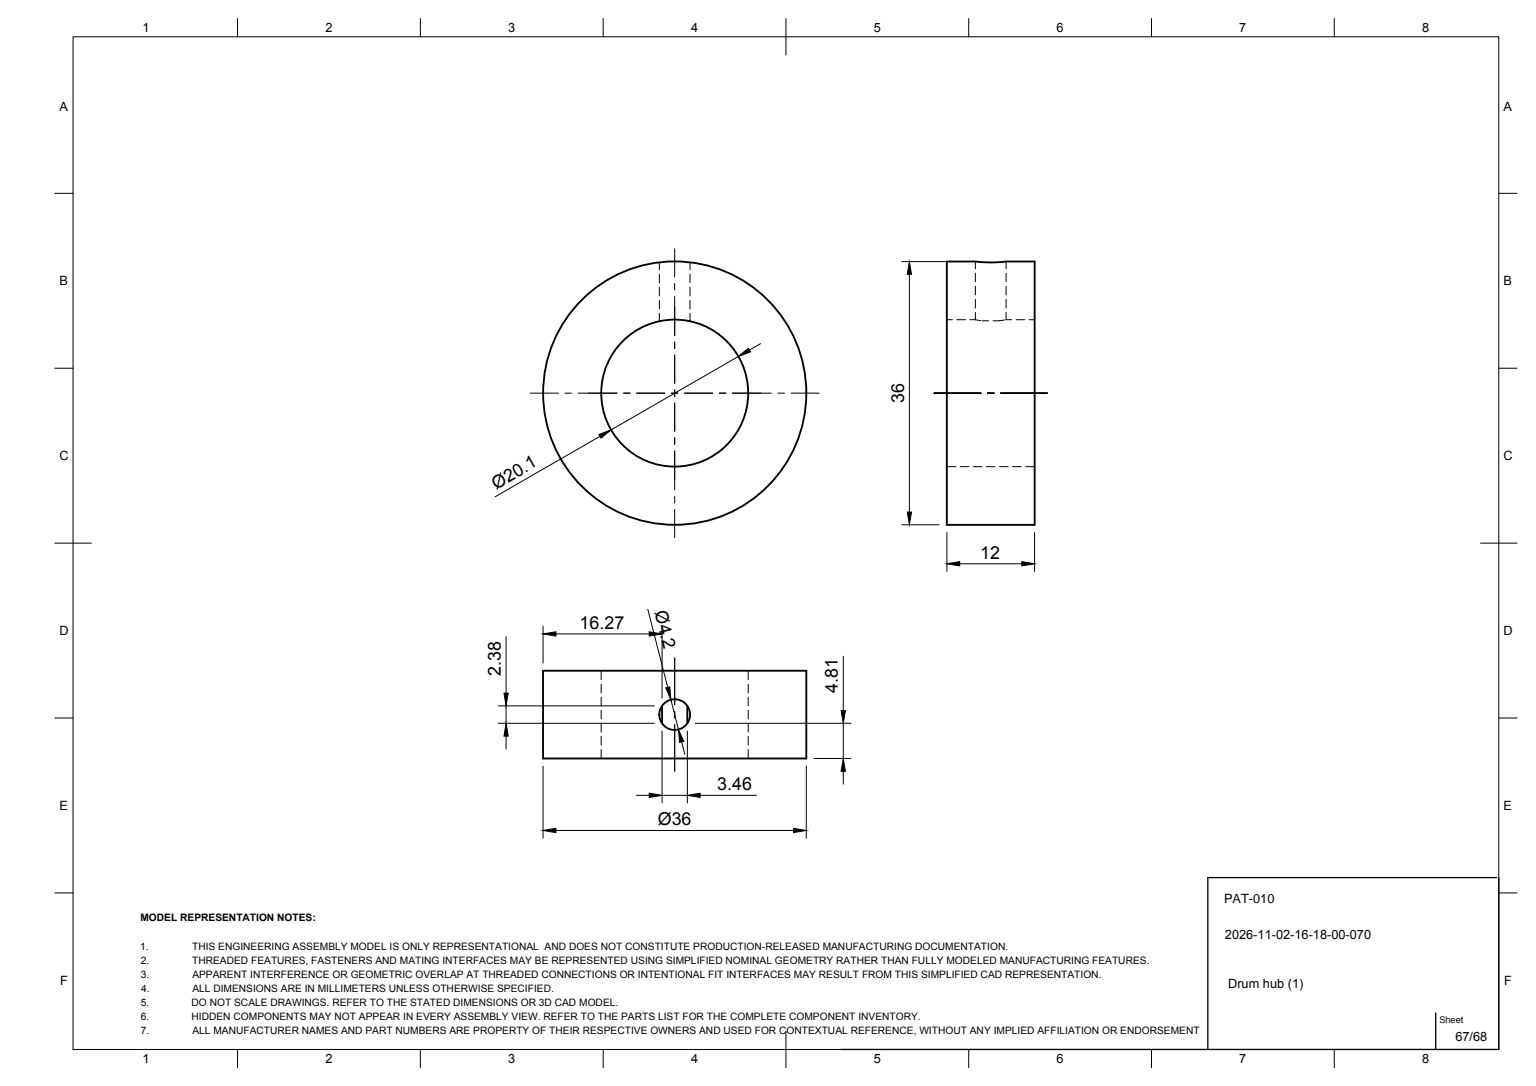
ISO-10303-21;
HEADER;
/* Generated by software containing ST-Developer
 * from STEP Tools, Inc. (www.steptools.com) 
 */

FILE_DESCRIPTION(
/* description */ ('Belt conveyor head drive unit'),
/* implementation_level */ '2;1');

FILE_NAME(
/* name */ 'Drum hub (1).step',
/* time_stamp */ '2026-10-28T03:26:19-07:00',
/* author */ (''),
/* organization */ (''),
/* preprocessor_version */ 'ST-DEVELOPER v20.2',
/* originating_system */ 'Autodesk Translation Framework v15.17.0.0',
/* authorisation */ '');

FILE_SCHEMA (('AUTOMOTIVE_DESIGN { 1 0 10303 214 3 1 1 }'));
ENDSEC;

DATA;
#10=MECHANICAL_DESIGN_GEOMETRIC_PRESENTATION_REPRESENTATION('',(#928),#27069);
#619=B_SPLINE_CURVE_WITH_KNOTS('',3,(#25750,#25751,#25752,#25753,#25754,
#25755,#25756,#25757,#25758,#25759,#25760,#25761,#25762,#25763),
 .UNSPECIFIED.,.F.,.F.,(4,2,2,2,2,2,4),(0.756005737987017,0.793568827564644,
0.872922520054199,0.952276212543754,1.03162990503331,1.11098359752286,1.1485466871005),
 .UNSPECIFIED.);
#620=B_SPLINE_CURVE_WITH_KNOTS('',3,(#25769,#25770,#25771,#25772,#25773,
#25774,#25775,#25776,#25777,#25778,#25779,#25780,#25781,#25782,#25783,#25784,
#25785,#25786),.UNSPECIFIED.,.F.,.F.,(4,2,2,2,2,2,2,2,4),(0.,0.0791819055472362,
0.158363811094472,0.237545215630595,0.316726620166717,0.395908024702839,
0.475089429238961,0.554271334786197,0.633453240333433),.UNSPECIFIED.);
#621=B_SPLINE_CURVE_WITH_KNOTS('',3,(#25787,#25788,#25789,#25790,#25791,
#25792,#25793,#25794,#25795,#25796,#25797,#25798,#25799,#25800,#25801,#25802,
#25803,#25804),.UNSPECIFIED.,.F.,.F.,(4,2,2,2,2,2,2,2,4),(0.633453240333433,
0.71263514588067,0.791817051427906,0.870998455964028,0.95017986050015,1.02936126503627,
1.10854266957239,1.18772457511963,1.26690648066687),.UNSPECIFIED.);
#622=B_SPLINE_CURVE_WITH_KNOTS('',3,(#25807,#25808,#25809,#25810,#25811,
#25812,#25813,#25814,#25815,#25816,#25817,#25818,#25819,#25820),
 .UNSPECIFIED.,.F.,.F.,(4,2,2,2,2,2,4),(0.121154929624508,0.158718019202141,
0.238071711691696,0.317425404181251,0.396779096670806,0.476132789160361,
0.513695878737978),.UNSPECIFIED.);
#774=SHAPE_REPRESENTATION_RELATIONSHIP('SRR','None',#27423,#843);
#843=ADVANCED_BREP_SHAPE_REPRESENTATION('',(#1009),#27065);
#928=STYLED_ITEM('',(#27783),#1009);
#1009=MANIFOLD_SOLID_BREP('Body1',#13797);
#1260=FACE_BOUND('',#3356,.T.);
#1261=FACE_BOUND('',#3358,.T.);
#1262=FACE_BOUND('',#3360,.T.);
#1263=FACE_BOUND('',#3362,.T.);
#1604=PLANE('',#16002);
#1605=PLANE('',#16007);
#1606=PLANE('',#16014);
#1607=PLANE('',#16015);
#2304=FACE_OUTER_BOUND('',#3352,.T.);
#2305=FACE_OUTER_BOUND('',#3353,.T.);
#2306=FACE_OUTER_BOUND('',#3354,.T.);
#2307=FACE_OUTER_BOUND('',#3355,.T.);
#2308=FACE_OUTER_BOUND('',#3357,.T.);
#2309=FACE_OUTER_BOUND('',#3359,.T.);
#2310=FACE_OUTER_BOUND('',#3361,.T.);
#3352=EDGE_LOOP('',(#11826,#11827));
#3353=EDGE_LOOP('',(#11828,#11829,#11830,#11831,#11832,#11833,#11834,#11835,
#11836));
#3354=EDGE_LOOP('',(#11837,#11838,#11839));
#3355=EDGE_LOOP('',(#11840,#11841,#11842,#11843));
#3356=EDGE_LOOP('',(#11844,#11845,#11846,#11847));
#3357=EDGE_LOOP('',(#11848,#11849,#11850,#11851));
#3358=EDGE_LOOP('',(#11852,#11853));
#3359=EDGE_LOOP('',(#11854));
#3360=EDGE_LOOP('',(#11855));
#3361=EDGE_LOOP('',(#11856));
#3362=EDGE_LOOP('',(#11857));
#4150=LINE('',#25746,#4942);
#4151=LINE('',#25767,#4943);
#4152=LINE('',#25822,#4944);
#4153=LINE('',#25827,#4945);
#4154=LINE('',#25833,#4946);
#4942=VECTOR('',#19968,1.);
#4943=VECTOR('',#19975,0.21);
#4944=VECTOR('',#19980,1.);
#4945=VECTOR('',#19985,1.005);
#4946=VECTOR('',#19992,1.8);
#5766=CIRCLE('',#16003,0.21);
#5767=CIRCLE('',#16005,0.21);
#5768=CIRCLE('',#16006,0.21);
#5769=CIRCLE('',#16009,1.005);
#5770=CIRCLE('',#16010,1.005);
#5771=CIRCLE('',#16012,1.8);
#5772=CIRCLE('',#16013,1.8);
#6934=VERTEX_POINT('',#25744);
#6935=VERTEX_POINT('',#25745);
#6936=VERTEX_POINT('',#25749);
#6937=VERTEX_POINT('',#25764);
#6938=VERTEX_POINT('',#25766);
#6939=VERTEX_POINT('',#25768);
#6940=VERTEX_POINT('',#25805);
#6941=VERTEX_POINT('',#25824);
#6942=VERTEX_POINT('',#25826);
#6943=VERTEX_POINT('',#25830);
#6944=VERTEX_POINT('',#25832);
#8605=EDGE_CURVE('',#6934,#6935,#4150,.T.);
#8606=EDGE_CURVE('',#6934,#6935,#5766,.T.);
#8607=EDGE_CURVE('',#6936,#6934,#619,.T.);
#8608=EDGE_CURVE('',#6937,#6936,#5767,.T.);
#8609=EDGE_CURVE('',#6937,#6938,#4151,.T.);
#8610=EDGE_CURVE('',#6939,#6938,#620,.T.);
#8611=EDGE_CURVE('',#6938,#6939,#621,.T.);
#8612=EDGE_CURVE('',#6940,#6937,#5768,.T.);
#8613=EDGE_CURVE('',#6935,#6940,#622,.T.);
#8614=EDGE_CURVE('',#6940,#6936,#4152,.T.);
#8615=EDGE_CURVE('',#6941,#6941,#5769,.T.);
#8616=EDGE_CURVE('',#6941,#6942,#4153,.T.);
#8617=EDGE_CURVE('',#6942,#6942,#5770,.T.);
#8618=EDGE_CURVE('',#6943,#6943,#5771,.T.);
#8619=EDGE_CURVE('',#6943,#6944,#4154,.T.);
#8620=EDGE_CURVE('',#6944,#6944,#5772,.T.);
#11826=ORIENTED_EDGE('',*,*,#8605,.F.);
#11827=ORIENTED_EDGE('',*,*,#8606,.T.);
#11828=ORIENTED_EDGE('',*,*,#8607,.F.);
#11829=ORIENTED_EDGE('',*,*,#8608,.F.);
#11830=ORIENTED_EDGE('',*,*,#8609,.T.);
#11831=ORIENTED_EDGE('',*,*,#8610,.F.);
#11832=ORIENTED_EDGE('',*,*,#8611,.F.);
#11833=ORIENTED_EDGE('',*,*,#8609,.F.);
#11834=ORIENTED_EDGE('',*,*,#8612,.F.);
#11835=ORIENTED_EDGE('',*,*,#8613,.F.);
#11836=ORIENTED_EDGE('',*,*,#8606,.F.);
#11837=ORIENTED_EDGE('',*,*,#8614,.F.);
#11838=ORIENTED_EDGE('',*,*,#8612,.T.);
#11839=ORIENTED_EDGE('',*,*,#8608,.T.);
#11840=ORIENTED_EDGE('',*,*,#8615,.F.);
#11841=ORIENTED_EDGE('',*,*,#8616,.T.);
#11842=ORIENTED_EDGE('',*,*,#8617,.T.);
#11843=ORIENTED_EDGE('',*,*,#8616,.F.);
#11844=ORIENTED_EDGE('',*,*,#8613,.T.);
#11845=ORIENTED_EDGE('',*,*,#8614,.T.);
#11846=ORIENTED_EDGE('',*,*,#8607,.T.);
#11847=ORIENTED_EDGE('',*,*,#8605,.T.);
#11848=ORIENTED_EDGE('',*,*,#8618,.F.);
#11849=ORIENTED_EDGE('',*,*,#8619,.T.);
#11850=ORIENTED_EDGE('',*,*,#8620,.T.);
#11851=ORIENTED_EDGE('',*,*,#8619,.F.);
#11852=ORIENTED_EDGE('',*,*,#8610,.T.);
#11853=ORIENTED_EDGE('',*,*,#8611,.T.);
#11854=ORIENTED_EDGE('',*,*,#8618,.T.);
#11855=ORIENTED_EDGE('',*,*,#8615,.T.);
#11856=ORIENTED_EDGE('',*,*,#8620,.F.);
#11857=ORIENTED_EDGE('',*,*,#8617,.F.);
#12818=CYLINDRICAL_SURFACE('',#16004,0.21);
#12819=CYLINDRICAL_SURFACE('',#16008,1.005);
#12820=CYLINDRICAL_SURFACE('',#16011,1.8);
#13583=ADVANCED_FACE('',(#2304),#1604,.T.);
#13584=ADVANCED_FACE('',(#2305),#12818,.F.);
#13585=ADVANCED_FACE('',(#2306),#1605,.T.);
#13586=ADVANCED_FACE('',(#2307,#1260),#12819,.F.);
#13587=ADVANCED_FACE('',(#2308,#1261),#12820,.T.);
#13588=ADVANCED_FACE('',(#2309,#1262),#1606,.T.);
#13589=ADVANCED_FACE('',(#2310,#1263),#1607,.F.);
#13797=CLOSED_SHELL('',(#13583,#13584,#13585,#13586,#13587,#13588,#13589));
#16001=AXIS2_PLACEMENT_3D('',#25742,#19964,#19965);
#16002=AXIS2_PLACEMENT_3D('',#25743,#19966,#19967);
#16003=AXIS2_PLACEMENT_3D('',#25747,#19969,#19970);
#16004=AXIS2_PLACEMENT_3D('',#25748,#19971,#19972);
#16005=AXIS2_PLACEMENT_3D('',#25765,#19973,#19974);
#16006=AXIS2_PLACEMENT_3D('',#25806,#19976,#19977);
#16007=AXIS2_PLACEMENT_3D('',#25821,#19978,#19979);
#16008=AXIS2_PLACEMENT_3D('',#25823,#19981,#19982);
#16009=AXIS2_PLACEMENT_3D('',#25825,#19983,#19984);
#16010=AXIS2_PLACEMENT_3D('',#25828,#19986,#19987);
#16011=AXIS2_PLACEMENT_3D('',#25829,#19988,#19989);
#16012=AXIS2_PLACEMENT_3D('',#25831,#19990,#19991);
#16013=AXIS2_PLACEMENT_3D('',#25834,#19993,#19994);
#16014=AXIS2_PLACEMENT_3D('',#25835,#19995,#19996);
#16015=AXIS2_PLACEMENT_3D('',#25836,#19997,#19998);
#19964=DIRECTION('axis',(0.,0.,1.));
#19965=DIRECTION('refdir',(1.,0.,0.));
#19966=DIRECTION('center_axis',(0.,0.,1.));
#19967=DIRECTION('ref_axis',(1.,0.,0.));
#19968=DIRECTION('',(0.,1.,0.));
#19969=DIRECTION('center_axis',(0.,0.,1.));
#19970=DIRECTION('ref_axis',(1.,0.,0.));
#19971=DIRECTION('center_axis',(0.,0.,1.));
#19972=DIRECTION('ref_axis',(1.,0.,0.));
#19973=DIRECTION('center_axis',(0.,0.,1.));
#19974=DIRECTION('ref_axis',(1.,0.,0.));
#19975=DIRECTION('',(0.,0.,1.));
#19976=DIRECTION('center_axis',(0.,0.,1.));
#19977=DIRECTION('ref_axis',(1.,0.,0.));
#19978=DIRECTION('center_axis',(0.,0.,1.));
#19979=DIRECTION('ref_axis',(1.,0.,0.));
#19980=DIRECTION('',(0.,-1.,0.));
#19981=DIRECTION('center_axis',(0.,1.,0.));
#19982=DIRECTION('ref_axis',(1.,0.,0.));
#19983=DIRECTION('center_axis',(0.,-1.,0.));
#19984=DIRECTION('ref_axis',(1.,0.,0.));
#19985=DIRECTION('',(0.,-1.,0.));
#19986=DIRECTION('center_axis',(0.,-1.,0.));
#19987=DIRECTION('ref_axis',(1.,0.,0.));
#19988=DIRECTION('center_axis',(0.,1.,0.));
#19989=DIRECTION('ref_axis',(1.,0.,0.));
#19990=DIRECTION('center_axis',(0.,1.,0.));
#19991=DIRECTION('ref_axis',(1.,0.,0.));
#19992=DIRECTION('',(0.,-1.,0.));
#19993=DIRECTION('center_axis',(0.,1.,0.));
#19994=DIRECTION('ref_axis',(1.,0.,0.));
#19995=DIRECTION('center_axis',(0.,1.,0.));
#19996=DIRECTION('ref_axis',(1.,0.,0.));
#19997=DIRECTION('center_axis',(0.,1.,0.));
#19998=DIRECTION('ref_axis',(1.,0.,0.));
#25742=CARTESIAN_POINT('',(0.,0.,0.));
#25743=CARTESIAN_POINT('Origin',(6.97091003018116,36.4,7.99));
#25744=CARTESIAN_POINT('',(7.14389846910121,36.2809411910021,7.99));
#25745=CARTESIAN_POINT('',(7.14389846910121,36.5190588089979,7.99));
#25746=CARTESIAN_POINT('',(7.14389846910121,35.8,7.99));
#25747=CARTESIAN_POINT('Origin',(6.97091003018116,36.4,7.99));
#25748=CARTESIAN_POINT('Origin',(6.97091003018116,36.4,7.99));
#25749=CARTESIAN_POINT('',(6.7979215912611,36.2809411910021,7.99));
#25750=CARTESIAN_POINT('Ctrl Pts',(6.7979215912611,36.2809411910021,7.99));
#25751=CARTESIAN_POINT('Ctrl Pts',(6.80531516486984,36.2701985776047,7.99129192197638));
#25752=CARTESIAN_POINT('Ctrl Pts',(6.81361289145555,36.2603122906273,7.99265394943905));
#25753=CARTESIAN_POINT('Ctrl Pts',(6.84101795633608,36.2329072257467,7.9967480843909));
#25754=CARTESIAN_POINT('Ctrl Pts',(6.86457986242187,36.216757943667,7.99969589327637));
#25755=CARTESIAN_POINT('Ctrl Pts',(6.91629712554875,36.1953022060351,8.00385029472357));
#25756=CARTESIAN_POINT('Ctrl Pts',(6.9444587993513,36.19,8.005));
#25757=CARTESIAN_POINT('Ctrl Pts',(6.99736126101101,36.19,8.005));
#25758=CARTESIAN_POINT('Ctrl Pts',(7.02552293481357,36.1953022060351,8.00385029472357));
#25759=CARTESIAN_POINT('Ctrl Pts',(7.07724019794044,36.216757943667,7.99969589327637));
#25760=CARTESIAN_POINT('Ctrl Pts',(7.10080210402623,36.2329072257467,7.9967480843909));
#25761=CARTESIAN_POINT('Ctrl Pts',(7.12820716890676,36.2603122906273,7.99265394943905));
#25762=CARTESIAN_POINT('Ctrl Pts',(7.13650489549247,36.2701985776047,7.99129192197638));
#25763=CARTESIAN_POINT('Ctrl Pts',(7.14389846910121,36.2809411910021,7.99));
#25764=CARTESIAN_POINT('',(6.76091003018116,36.4,7.99));
#25765=CARTESIAN_POINT('Origin',(6.97091003018116,36.4,7.99));
#25766=CARTESIAN_POINT('',(6.76091003018116,36.4,8.78770802985275));
#25767=CARTESIAN_POINT('',(6.76091003018116,36.4,7.99));
#25768=CARTESIAN_POINT('',(7.18091003018116,36.4,8.78770802985275));
#25769=CARTESIAN_POINT('Ctrl Pts',(7.18091003018116,36.4,8.78770802985275));
#25770=CARTESIAN_POINT('Ctrl Pts',(7.18091003018116,36.3736060314843,8.78770802985275));
#25771=CARTESIAN_POINT('Ctrl Pts',(7.17563026313289,36.345469345566,8.78835284034214));
#25772=CARTESIAN_POINT('Ctrl Pts',(7.15419155416006,36.293736883974,8.79067700538683));
#25773=CARTESIAN_POINT('Ctrl Pts',(7.13803391906352,36.270139040784,8.79232226897314));
#25774=CARTESIAN_POINT('Ctrl Pts',(7.10077110728482,36.2328762290053,8.79540680803063));
#25775=CARTESIAN_POINT('Ctrl Pts',(7.07717321270923,36.2167185016358,8.79704717240673));
#25776=CARTESIAN_POINT('Ctrl Pts',(7.02544057769236,36.1952797246826,8.79936011492601));
#25777=CARTESIAN_POINT('Ctrl Pts',(6.9973038316932,36.19,8.8));
#25778=CARTESIAN_POINT('Ctrl Pts',(6.94451622866912,36.19,8.8));
#25779=CARTESIAN_POINT('Ctrl Pts',(6.91637948266995,36.1952797246826,8.79936011492601));
#25780=CARTESIAN_POINT('Ctrl Pts',(6.86464684765309,36.2167185016358,8.79704717240673));
#25781=CARTESIAN_POINT('Ctrl Pts',(6.84104895307749,36.2328762290053,8.79540680803063));
#25782=CARTESIAN_POINT('Ctrl Pts',(6.80378614129879,36.270139040784,8.79232226897314));
#25783=CARTESIAN_POINT('Ctrl Pts',(6.78762850620225,36.293736883974,8.79067700538683));
#25784=CARTESIAN_POINT('Ctrl Pts',(6.76618979722943,36.345469345566,8.78835284034214));
#25785=CARTESIAN_POINT('Ctrl Pts',(6.76091003018116,36.3736060314843,8.78770802985275));
#25786=CARTESIAN_POINT('Ctrl Pts',(6.76091003018116,36.4,8.78770802985275));
#25787=CARTESIAN_POINT('Ctrl Pts',(6.76091003018116,36.4,8.78770802985275));
#25788=CARTESIAN_POINT('Ctrl Pts',(6.76091003018116,36.4263939685157,8.78770802985275));
#25789=CARTESIAN_POINT('Ctrl Pts',(6.76618979722943,36.454530654434,8.78835284034214));
#25790=CARTESIAN_POINT('Ctrl Pts',(6.78762850620225,36.506263116026,8.79067700538683));
#25791=CARTESIAN_POINT('Ctrl Pts',(6.80378614129879,36.529860959216,8.79232226897314));
#25792=CARTESIAN_POINT('Ctrl Pts',(6.84104895307749,36.5671237709947,8.79540680803063));
#25793=CARTESIAN_POINT('Ctrl Pts',(6.86464684765309,36.5832814983642,8.79704717240673));
#25794=CARTESIAN_POINT('Ctrl Pts',(6.91637948266995,36.6047202753174,8.79936011492601));
#25795=CARTESIAN_POINT('Ctrl Pts',(6.94451622866912,36.61,8.8));
#25796=CARTESIAN_POINT('Ctrl Pts',(6.9973038316932,36.61,8.8));
#25797=CARTESIAN_POINT('Ctrl Pts',(7.02544057769236,36.6047202753174,8.79936011492601));
#25798=CARTESIAN_POINT('Ctrl Pts',(7.07717321270923,36.5832814983642,8.79704717240673));
#25799=CARTESIAN_POINT('Ctrl Pts',(7.10077110728482,36.5671237709947,8.79540680803063));
#25800=CARTESIAN_POINT('Ctrl Pts',(7.13803391906352,36.529860959216,8.79232226897314));
#25801=CARTESIAN_POINT('Ctrl Pts',(7.15419155416006,36.506263116026,8.79067700538683));
#25802=CARTESIAN_POINT('Ctrl Pts',(7.17563026313288,36.454530654434,8.78835284034214));
#25803=CARTESIAN_POINT('Ctrl Pts',(7.18091003018116,36.4263939685157,8.78770802985275));
#25804=CARTESIAN_POINT('Ctrl Pts',(7.18091003018116,36.4,8.78770802985275));
#25805=CARTESIAN_POINT('',(6.7979215912611,36.5190588089979,7.99));
#25806=CARTESIAN_POINT('Origin',(6.97091003018116,36.4,7.99));
#25807=CARTESIAN_POINT('Ctrl Pts',(7.14389846910122,36.5190588089979,7.99));
#25808=CARTESIAN_POINT('Ctrl Pts',(7.13650489549247,36.5298014223953,7.99129192197638));
#25809=CARTESIAN_POINT('Ctrl Pts',(7.12820716890676,36.5396877093727,7.99265394943905));
#25810=CARTESIAN_POINT('Ctrl Pts',(7.10080210402623,36.5670927742533,7.9967480843909));
#25811=CARTESIAN_POINT('Ctrl Pts',(7.07724019794044,36.5832420563329,7.99969589327637));
#25812=CARTESIAN_POINT('Ctrl Pts',(7.02552293481357,36.6046977939649,8.00385029472357));
#25813=CARTESIAN_POINT('Ctrl Pts',(6.99736126101101,36.61,8.005));
#25814=CARTESIAN_POINT('Ctrl Pts',(6.9444587993513,36.61,8.005));
#25815=CARTESIAN_POINT('Ctrl Pts',(6.91629712554875,36.6046977939649,8.00385029472357));
#25816=CARTESIAN_POINT('Ctrl Pts',(6.86457986242187,36.5832420563329,7.99969589327637));
#25817=CARTESIAN_POINT('Ctrl Pts',(6.84101795633608,36.5670927742533,7.9967480843909));
#25818=CARTESIAN_POINT('Ctrl Pts',(6.81361289145555,36.5396877093727,7.99265394943905));
#25819=CARTESIAN_POINT('Ctrl Pts',(6.80531516486984,36.5298014223953,7.99129192197638));
#25820=CARTESIAN_POINT('Ctrl Pts',(6.7979215912611,36.5190588089979,7.99));
#25821=CARTESIAN_POINT('Origin',(6.97091003018116,36.4,7.99));
#25822=CARTESIAN_POINT('',(6.7979215912611,35.8,7.99));
#25823=CARTESIAN_POINT('Origin',(6.97091003018116,35.8,7.));
#25824=CARTESIAN_POINT('',(5.96591003018116,37.,7.));
#25825=CARTESIAN_POINT('Origin',(6.97091003018116,37.,7.));
#25826=CARTESIAN_POINT('',(5.96591003018116,35.8,7.));
#25827=CARTESIAN_POINT('',(5.96591003018116,35.8,7.));
#25828=CARTESIAN_POINT('Origin',(6.97091003018116,35.8,7.));
#25829=CARTESIAN_POINT('Origin',(6.97091003018116,35.8,7.));
#25830=CARTESIAN_POINT('',(5.17091003018116,37.,7.));
#25831=CARTESIAN_POINT('Origin',(6.97091003018116,37.,7.));
#25832=CARTESIAN_POINT('',(5.17091003018116,35.8,7.));
#25833=CARTESIAN_POINT('',(5.17091003018116,35.8,7.));
#25834=CARTESIAN_POINT('Origin',(6.97091003018116,35.8,7.));
#25835=CARTESIAN_POINT('Origin',(6.97091003018116,37.,7.));
#25836=CARTESIAN_POINT('Origin',(6.97091003018116,35.8,7.));
#26988=UNCERTAINTY_MEASURE_WITH_UNIT(LENGTH_MEASURE(0.001),#27070,
'DISTANCE_ACCURACY_VALUE',
'Maximum model space distance between geometric entities at asserted c
onnectivities');
#26992=UNCERTAINTY_MEASURE_WITH_UNIT(LENGTH_MEASURE(0.001),#27070,
'DISTANCE_ACCURACY_VALUE',
'Maximum model space distance between geometric entities at asserted c
onnectivities');
#27065=(
GEOMETRIC_REPRESENTATION_CONTEXT(3)
GLOBAL_UNCERTAINTY_ASSIGNED_CONTEXT((#26988))
GLOBAL_UNIT_ASSIGNED_CONTEXT((#27070,#27072,#27073))
REPRESENTATION_CONTEXT('','3D')
);
#27069=(
GEOMETRIC_REPRESENTATION_CONTEXT(3)
GLOBAL_UNCERTAINTY_ASSIGNED_CONTEXT((#26992))
GLOBAL_UNIT_ASSIGNED_CONTEXT((#27070,#27072,#27073))
REPRESENTATION_CONTEXT('','3D')
);
#27070=(
LENGTH_UNIT()
NAMED_UNIT(*)
SI_UNIT(.CENTI.,.METRE.)
);
#27072=(
NAMED_UNIT(*)
PLANE_ANGLE_UNIT()
SI_UNIT($,.RADIAN.)
);
#27073=(
NAMED_UNIT(*)
SI_UNIT($,.STERADIAN.)
SOLID_ANGLE_UNIT()
);
#27146=SHAPE_DEFINITION_REPRESENTATION(#27234,#27423);
#27234=PRODUCT_DEFINITION_SHAPE('',$,#27500);
#27423=SHAPE_REPRESENTATION('',(#16001),#27065);
#27427=PRODUCT_DEFINITION_CONTEXT('part definition',#27657,'design');
#27500=PRODUCT_DEFINITION('Drum hub (1)','Drum hub (1)',#27576,#27427);
#27576=PRODUCT_DEFINITION_FORMATION('',$,#27731);
#27657=APPLICATION_CONTEXT(
'Core Data for Automotive Mechanical Design Process');
#27658=PRODUCT_CONTEXT('part definition',#27657,'mechanical');
#27731=PRODUCT('Drum hub (1)','Drum hub (1)','Drum hub (1)',(#27658));
#27777=COLOUR_RGB('Light Blue',0.38,0.62,0.78);
#27778=FILL_AREA_STYLE_COLOUR('',#27777);
#27779=FILL_AREA_STYLE('',(#27778));
#27780=SURFACE_STYLE_FILL_AREA(#27779);
#27781=SURFACE_SIDE_STYLE('',(#27780));
#27782=SURFACE_STYLE_USAGE(.BOTH.,#27781);
#27783=PRESENTATION_STYLE_ASSIGNMENT((#27782));
ENDSEC;
END-ISO-10303-21;
